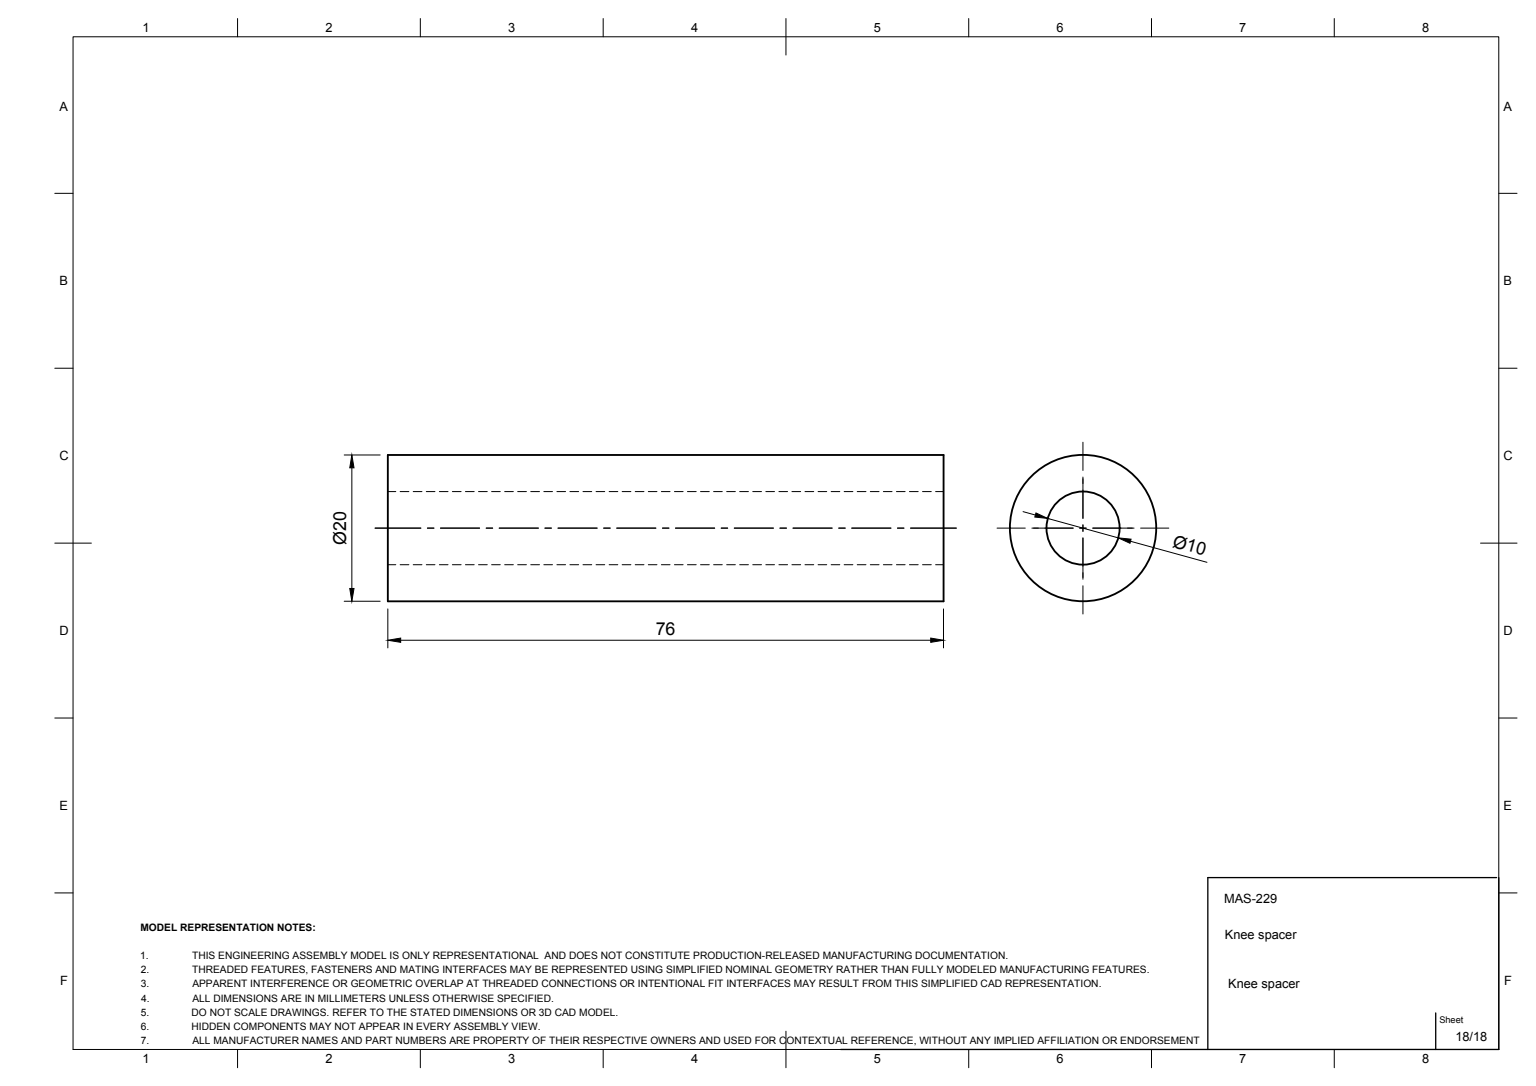
ISO-10303-21;
HEADER;
/* Generated by software containing ST-Developer
 * from STEP Tools, Inc. (www.steptools.com) 
 */

FILE_DESCRIPTION(
/* description */ ('Independently dimensioned six-bar single-leg walking-linkage demonstr
ator. Whole-mm20 crank,60 upper rocker,80/120 ternary coupler,120 lowe
r rocker,140 knee pitch and260 toe reach; ground pivots0/0,60/0,40/60.
 Seven native revolutes close both loops. Four reused native library f
amilies, fully retained shared pins and layered real spacer stacks, bo
nded rubber toe. Benchtop reference mechanism; no complete vehicle, lo
ad, gait stability, adhesive, weld, fit or life rating.'),
/* implementation_level */ '2;1');

FILE_NAME(
/* name */ 'Knee spacer.step',
/* time_stamp */ '2026-11-09T20:33:14-08:00',
/* author */ (''),
/* organization */ (''),
/* preprocessor_version */ 'ST-DEVELOPER v20.2',
/* originating_system */ 'Autodesk Translation Framework v15.17.0.0',
/* authorisation */ '');

FILE_SCHEMA (('AUTOMOTIVE_DESIGN { 1 0 10303 214 3 1 1 }'));
ENDSEC;

DATA;
#10=MECHANICAL_DESIGN_GEOMETRIC_PRESENTATION_REPRESENTATION('',(#268),#4048);
#232=SHAPE_REPRESENTATION_RELATIONSHIP('SRR','None',#4156,#250);
#250=ADVANCED_BREP_SHAPE_REPRESENTATION('',(#286),#4043);
#268=STYLED_ITEM('',(#4253),#286);
#286=MANIFOLD_SOLID_BREP('Body1',#2157);
#339=FACE_BOUND('',#691,.T.);
#340=FACE_BOUND('',#693,.T.);
#400=PLANE('',#2571);
#401=PLANE('',#2572);
#514=FACE_OUTER_BOUND('',#688,.T.);
#515=FACE_OUTER_BOUND('',#689,.T.);
#516=FACE_OUTER_BOUND('',#690,.T.);
#517=FACE_OUTER_BOUND('',#692,.T.);
#688=EDGE_LOOP('',(#1879,#1880,#1881,#1882));
#689=EDGE_LOOP('',(#1883,#1884,#1885,#1886));
#690=EDGE_LOOP('',(#1887));
#691=EDGE_LOOP('',(#1888));
#692=EDGE_LOOP('',(#1889));
#693=EDGE_LOOP('',(#1890));
#831=LINE('',#3861,#956);
#832=LINE('',#3867,#957);
#956=VECTOR('',#3190,5.);
#957=VECTOR('',#3197,10.);
#1064=CIRCLE('',#2566,5.);
#1065=CIRCLE('',#2567,5.);
#1066=CIRCLE('',#2569,10.);
#1067=CIRCLE('',#2570,10.);
#1218=VERTEX_POINT('',#3858);
#1219=VERTEX_POINT('',#3860);
#1220=VERTEX_POINT('',#3864);
#1221=VERTEX_POINT('',#3866);
#1443=EDGE_CURVE('',#1218,#1218,#1064,.T.);
#1444=EDGE_CURVE('',#1218,#1219,#831,.T.);
#1445=EDGE_CURVE('',#1219,#1219,#1065,.T.);
#1446=EDGE_CURVE('',#1220,#1220,#1066,.T.);
#1447=EDGE_CURVE('',#1220,#1221,#832,.T.);
#1448=EDGE_CURVE('',#1221,#1221,#1067,.T.);
#1879=ORIENTED_EDGE('',*,*,#1443,.F.);
#1880=ORIENTED_EDGE('',*,*,#1444,.T.);
#1881=ORIENTED_EDGE('',*,*,#1445,.T.);
#1882=ORIENTED_EDGE('',*,*,#1444,.F.);
#1883=ORIENTED_EDGE('',*,*,#1446,.F.);
#1884=ORIENTED_EDGE('',*,*,#1447,.T.);
#1885=ORIENTED_EDGE('',*,*,#1448,.T.);
#1886=ORIENTED_EDGE('',*,*,#1447,.F.);
#1887=ORIENTED_EDGE('',*,*,#1446,.T.);
#1888=ORIENTED_EDGE('',*,*,#1443,.T.);
#1889=ORIENTED_EDGE('',*,*,#1448,.F.);
#1890=ORIENTED_EDGE('',*,*,#1445,.F.);
#2006=CYLINDRICAL_SURFACE('',#2565,5.);
#2007=CYLINDRICAL_SURFACE('',#2568,10.);
#2117=ADVANCED_FACE('',(#514),#2006,.F.);
#2118=ADVANCED_FACE('',(#515),#2007,.T.);
#2119=ADVANCED_FACE('',(#516,#339),#400,.T.);
#2120=ADVANCED_FACE('',(#517,#340),#401,.F.);
#2157=CLOSED_SHELL('',(#2117,#2118,#2119,#2120));
#2564=AXIS2_PLACEMENT_3D('',#3856,#3184,#3185);
#2565=AXIS2_PLACEMENT_3D('',#3857,#3186,#3187);
#2566=AXIS2_PLACEMENT_3D('',#3859,#3188,#3189);
#2567=AXIS2_PLACEMENT_3D('',#3862,#3191,#3192);
#2568=AXIS2_PLACEMENT_3D('',#3863,#3193,#3194);
#2569=AXIS2_PLACEMENT_3D('',#3865,#3195,#3196);
#2570=AXIS2_PLACEMENT_3D('',#3868,#3198,#3199);
#2571=AXIS2_PLACEMENT_3D('',#3869,#3200,#3201);
#2572=AXIS2_PLACEMENT_3D('',#3870,#3202,#3203);
#3184=DIRECTION('axis',(0.,0.,1.));
#3185=DIRECTION('refdir',(1.,0.,0.));
#3186=DIRECTION('center_axis',(0.,0.,1.));
#3187=DIRECTION('ref_axis',(1.,0.,0.));
#3188=DIRECTION('center_axis',(0.,0.,-1.));
#3189=DIRECTION('ref_axis',(1.,0.,0.));
#3190=DIRECTION('',(0.,0.,-1.));
#3191=DIRECTION('center_axis',(0.,0.,-1.));
#3192=DIRECTION('ref_axis',(1.,0.,0.));
#3193=DIRECTION('center_axis',(0.,0.,1.));
#3194=DIRECTION('ref_axis',(1.,0.,0.));
#3195=DIRECTION('center_axis',(0.,0.,1.));
#3196=DIRECTION('ref_axis',(1.,0.,0.));
#3197=DIRECTION('',(0.,0.,-1.));
#3198=DIRECTION('center_axis',(0.,0.,1.));
#3199=DIRECTION('ref_axis',(1.,0.,0.));
#3200=DIRECTION('center_axis',(0.,0.,1.));
#3201=DIRECTION('ref_axis',(1.,0.,0.));
#3202=DIRECTION('center_axis',(0.,0.,1.));
#3203=DIRECTION('ref_axis',(1.,0.,0.));
#3856=CARTESIAN_POINT('',(0.,0.,0.));
#3857=CARTESIAN_POINT('Origin',(0.,0.,0.));
#3858=CARTESIAN_POINT('',(-5.,-6.12323399573677E-16,76.));
#3859=CARTESIAN_POINT('Origin',(0.,0.,76.));
#3860=CARTESIAN_POINT('',(-5.,-6.12323399573677E-16,0.));
#3861=CARTESIAN_POINT('',(-5.,-6.12323399573677E-16,0.));
#3862=CARTESIAN_POINT('Origin',(0.,0.,0.));
#3863=CARTESIAN_POINT('Origin',(0.,0.,0.));
#3864=CARTESIAN_POINT('',(-10.,-1.22464679914735E-15,76.));
#3865=CARTESIAN_POINT('Origin',(0.,0.,76.));
#3866=CARTESIAN_POINT('',(-10.,-1.22464679914735E-15,0.));
#3867=CARTESIAN_POINT('',(-10.,-1.22464679914735E-15,0.));
#3868=CARTESIAN_POINT('Origin',(0.,0.,0.));
#3869=CARTESIAN_POINT('Origin',(0.,0.,76.));
#3870=CARTESIAN_POINT('Origin',(0.,0.,0.));
#4023=UNCERTAINTY_MEASURE_WITH_UNIT(LENGTH_MEASURE(0.01),#4049,
'DISTANCE_ACCURACY_VALUE',
'Maximum model space distance between geometric entities at asserted c
onnectivities');
#4028=UNCERTAINTY_MEASURE_WITH_UNIT(LENGTH_MEASURE(0.01),#4049,
'DISTANCE_ACCURACY_VALUE',
'Maximum model space distance between geometric entities at asserted c
onnectivities');
#4043=(
GEOMETRIC_REPRESENTATION_CONTEXT(3)
GLOBAL_UNCERTAINTY_ASSIGNED_CONTEXT((#4023))
GLOBAL_UNIT_ASSIGNED_CONTEXT((#4049,#4051,#4052))
REPRESENTATION_CONTEXT('','3D')
);
#4048=(
GEOMETRIC_REPRESENTATION_CONTEXT(3)
GLOBAL_UNCERTAINTY_ASSIGNED_CONTEXT((#4028))
GLOBAL_UNIT_ASSIGNED_CONTEXT((#4049,#4051,#4052))
REPRESENTATION_CONTEXT('','3D')
);
#4049=(
LENGTH_UNIT()
NAMED_UNIT(*)
SI_UNIT(.MILLI.,.METRE.)
);
#4051=(
NAMED_UNIT(*)
PLANE_ANGLE_UNIT()
SI_UNIT($,.RADIAN.)
);
#4052=(
NAMED_UNIT(*)
SI_UNIT($,.STERADIAN.)
SOLID_ANGLE_UNIT()
);
#4067=SHAPE_DEFINITION_REPRESENTATION(#4086,#4156);
#4086=PRODUCT_DEFINITION_SHAPE('',$,#4176);
#4156=SHAPE_REPRESENTATION('',(#2564),#4043);
#4161=PRODUCT_DEFINITION_CONTEXT('part definition',#4220,'design');
#4176=PRODUCT_DEFINITION('Knee spacer','Knee spacer',#4195,#4161);
#4195=PRODUCT_DEFINITION_FORMATION('',$,#4236);
#4220=APPLICATION_CONTEXT(
'Core Data for Automotive Mechanical Design Process');
#4221=PRODUCT_CONTEXT('part definition',#4220,'mechanical');
#4236=PRODUCT('Knee spacer','Knee spacer',$,(#4221));
#4253=PRESENTATION_STYLE_ASSIGNMENT((#4267));
#4267=SURFACE_STYLE_USAGE(.BOTH.,#4281);
#4281=SURFACE_SIDE_STYLE('',(#4295));
#4295=SURFACE_STYLE_FILL_AREA(#4309);
#4309=FILL_AREA_STYLE('Spacer gray',(#4323));
#4323=FILL_AREA_STYLE_COLOUR('Spacer gray',#4337);
#4337=COLOUR_RGB('Spacer gray',0.576470588235294,0.615686274509804,0.666666666666667);
ENDSEC;
END-ISO-10303-21;
